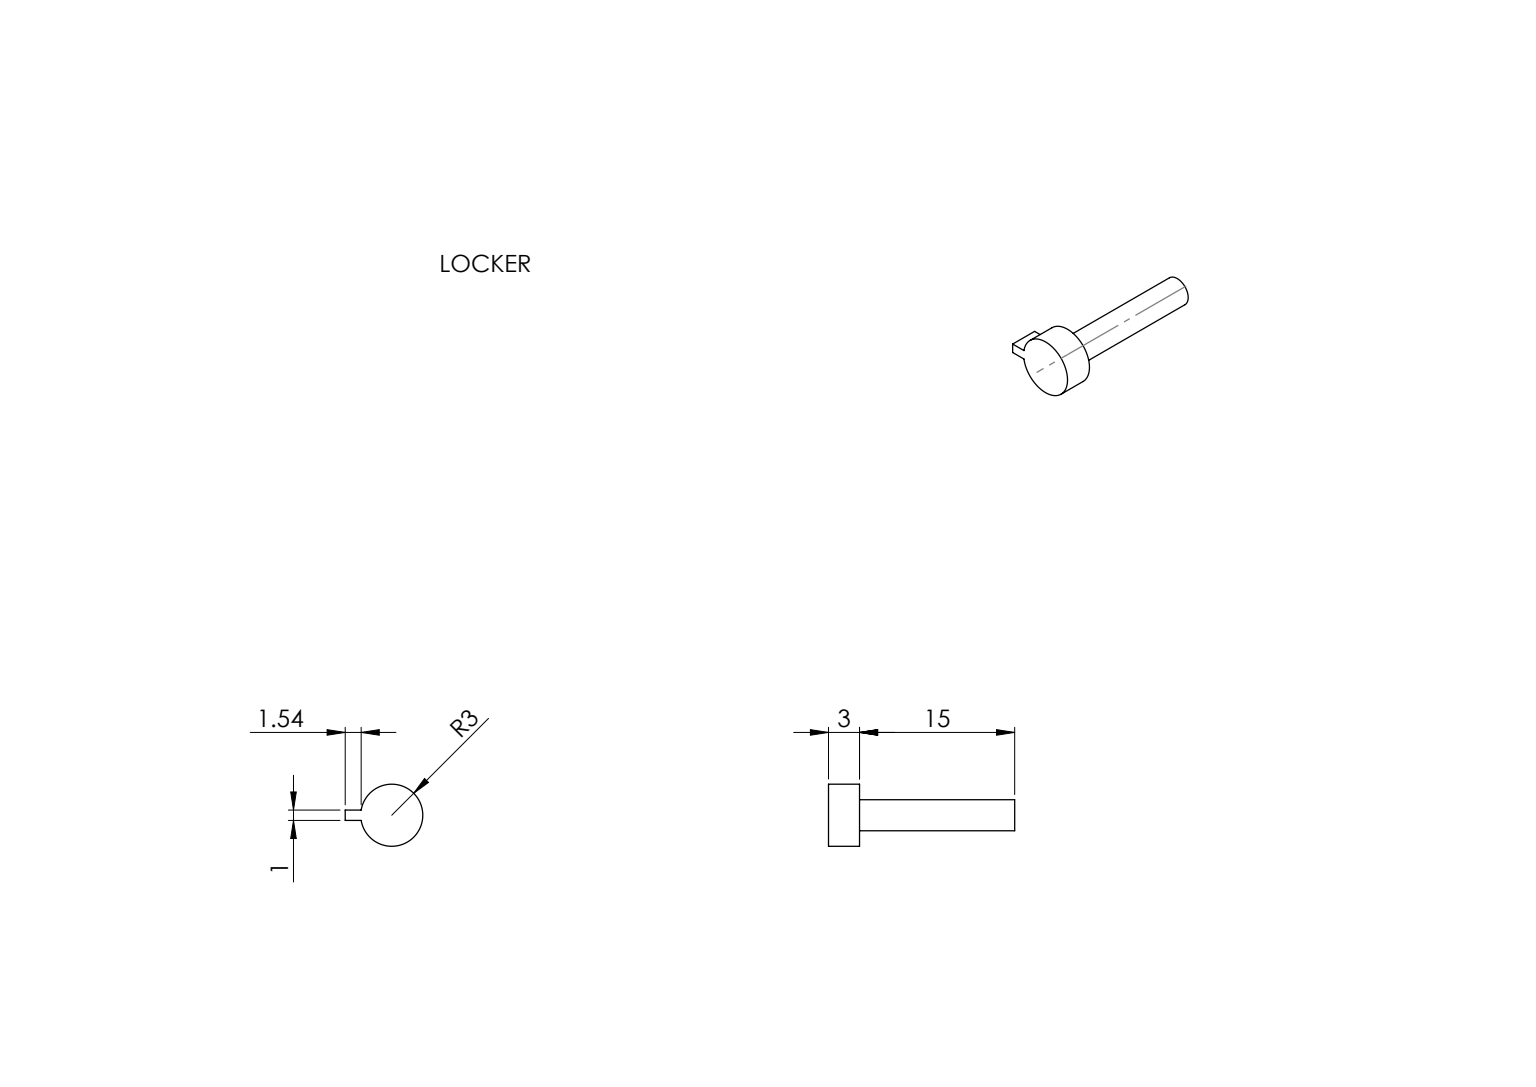
ISO-10303-21;
HEADER;
FILE_DESCRIPTION (('STEP AP214'),
    '1' );
FILE_NAME ('locker.step',
    '2026-10-08T12:30:53',
    ( '' ),
    ( '' ),
    'SwSTEP 2.0',
    'SolidWorks 2026',
    '' );
FILE_SCHEMA (( 'AUTOMOTIVE_DESIGN' ));
ENDSEC;

DATA;
#21=MECHANICAL_DESIGN_GEOMETRIC_PRESENTATION_REPRESENTATION('',(#419),#8834);
#84=LINE ( 'NONE', #11348, #8005 ) ;
#86=ORIENTED_EDGE ( 'NONE', *, *, #7277, .F. ) ;
#98=DIRECTION ( 'NONE',  ( -0.000000000000000000, 0.000000000000000000, 1.000000000000000000 ) ) ;
#220=PRODUCT ( 'locker', 'locker', '', ( #5871 ) ) ;
#374=( LENGTH_UNIT ( ) NAMED_UNIT ( * ) SI_UNIT ( .MILLI., .METRE. ) );
#389=VECTOR ( 'NONE', #4390, 1000.000000000000000 ) ;
#419=STYLED_ITEM ( 'NONE', ( #8733 ), #4375 ) ;
#434=SURFACE_STYLE_USAGE ( .BOTH. , #4112 ) ;
#484=CARTESIAN_POINT ( 'NONE',  ( -4.500000000000000888, 3.903127820947816751E-15, 0.000000000000000000 ) ) ;
#643=DIRECTION ( 'NONE',  ( -1.000000000000000000, -1.445602896647338917E-16, 0.000000000000000000 ) ) ;
#647=ADVANCED_FACE ( 'NONE', ( #2949 ), #10345, .T. ) ;
#766=CYLINDRICAL_SURFACE ( 'NONE', #2507, 1.500000000000000222 ) ;
#773=ORIENTED_EDGE ( 'NONE', *, *, #5743, .F. ) ;
#787=ORIENTED_EDGE ( 'NONE', *, *, #5743, .T. ) ;
#825=EDGE_CURVE ( 'NONE', #4657, #6571, #6084, .T. ) ;
#833=EDGE_CURVE ( 'NONE', #7905, #2790, #10011, .T. ) ;
#987=DIRECTION ( 'NONE',  ( -8.673617379884035472E-16, -1.000000000000000000, 0.000000000000000000 ) ) ;
#1034=CARTESIAN_POINT ( 'NONE',  ( 0.000000000000000000, 0.000000000000000000, 0.000000000000000000 ) ) ;
#1042=PLANE ( 'NONE',  #11528 ) ;
#1047=DIRECTION ( 'NONE',  ( -1.000000000000000000, -1.445602896647339163E-16, 0.000000000000000000 ) ) ;
#1166=CARTESIAN_POINT ( 'NONE',  ( 0.000000000000000000, 0.000000000000000000, 3.000000000000000000 ) ) ;
#1243=FACE_OUTER_BOUND ( 'NONE', #10896, .T. ) ;
#1269=LINE ( 'NONE', #4259, #1726 ) ;
#1297=DIRECTION ( 'NONE',  ( 1.445602896647339163E-16, -1.000000000000000000, 0.000000000000000000 ) ) ;
#1348=ORIENTED_EDGE ( 'NONE', *, *, #833, .F. ) ;
#1393=DIRECTION ( 'NONE',  ( -0.000000000000000000, 0.000000000000000000, 1.000000000000000000 ) ) ;
#1404=DIRECTION ( 'NONE',  ( -0.000000000000000000, -0.000000000000000000, 1.000000000000000000 ) ) ;
#1425=EDGE_CURVE ( 'NONE', #3560, #7905, #5417, .T. ) ;
#1470=ORIENTED_EDGE ( 'NONE', *, *, #3009, .F. ) ;
#1522=ORIENTED_EDGE ( 'NONE', *, *, #6465, .T. ) ;
#1551=DIRECTION ( 'NONE',  ( 0.000000000000000000, 0.000000000000000000, 1.000000000000000000 ) ) ;
#1580=EDGE_LOOP ( 'NONE', ( #3082, #9963, #2261, #1740 ) ) ;
#1644=EDGE_CURVE ( 'NONE', #4353, #2834, #9779, .T. ) ;
#1674=CARTESIAN_POINT ( 'NONE',  ( 0.000000000000000000, 0.000000000000000000, 0.000000000000000000 ) ) ;
#1688=VECTOR ( 'NONE', #1404, 1000.000000000000000 ) ;
#1726=VECTOR ( 'NONE', #5002, 1000.000000000000000 ) ;
#1737=ORIENTED_EDGE ( 'NONE', *, *, #3104, .F. ) ;
#1740=ORIENTED_EDGE ( 'NONE', *, *, #3104, .T. ) ;
#1741=PLANE ( 'NONE',  #6816 ) ;
#1843=ORIENTED_EDGE ( 'NONE', *, *, #3009, .T. ) ;
#1844=CARTESIAN_POINT ( 'NONE',  ( -4.500000000000000888, 3.903127820947816751E-15, 3.000000000000000000 ) ) ;
#1911=CARTESIAN_POINT ( 'NONE',  ( -2.958039891549808953, -0.4999999999999997780, 3.000000000000000000 ) ) ;
#2021=VERTEX_POINT ( 'NONE', #11151 ) ;
#2062=CARTESIAN_POINT ( 'NONE',  ( 0.000000000000000000, 0.000000000000000000, -15.00000000000000000 ) ) ;
#2072=CARTESIAN_POINT ( 'NONE',  ( -4.500000000000000000, 0.4999999999999998890, 3.000000000000000000 ) ) ;
#2077=ORIENTED_EDGE ( 'NONE', *, *, #1425, .F. ) ;
#2096=( NAMED_UNIT ( * ) SI_UNIT ( $, .STERADIAN. ) SOLID_ANGLE_UNIT ( ) );
#2102=ADVANCED_FACE ( 'NONE', ( #10529 ), #3991, .T. ) ;
#2146=DIRECTION ( 'NONE',  ( 1.000000000000000000, 0.000000000000000000, 0.000000000000000000 ) ) ;
#2154=SURFACE_STYLE_FILL_AREA ( #10536 ) ;
#2218=SHAPE_REPRESENTATION_RELATIONSHIP ( 'NONE' , 'NONE' ,  #8353, #2941 ) ;
#2261=ORIENTED_EDGE ( 'NONE', *, *, #1425, .T. ) ;
#2274=DIRECTION ( 'NONE',  ( 1.000000000000000000, 1.445602896647339163E-16, 0.000000000000000000 ) ) ;
#2407=AXIS2_PLACEMENT_3D ( 'NONE', #1034, #98, #3844 ) ;
#2486=DIRECTION ( 'NONE',  ( -1.000000000000000000, 0.000000000000000000, 0.000000000000000000 ) ) ;
#2507=AXIS2_PLACEMENT_3D ( 'NONE', #11053, #10008, #5371 ) ;
#2549=CARTESIAN_POINT ( 'NONE',  ( -4.500000000000000888, -0.5000000000000000000, 3.000000000000000000 ) ) ;
#2653=DIRECTION ( 'NONE',  ( 1.000000000000000000, 0.000000000000000000, 0.000000000000000000 ) ) ;
#2742=LINE ( 'NONE', #2931, #8579 ) ;
#2773=ADVANCED_FACE ( 'NONE', ( #6657 ), #1042, .T. ) ;
#2790=VERTEX_POINT ( 'NONE', #2072 ) ;
#2824=LINE ( 'NONE', #4658, #3000 ) ;
#2834=VERTEX_POINT ( 'NONE', #5988 ) ;
#2887=AXIS2_PLACEMENT_3D ( 'NONE', #9020, #4365, #11365 ) ;
#2931=CARTESIAN_POINT ( 'NONE',  ( -7.228014483236704444E-17, 0.5000000000000005551, 0.000000000000000000 ) ) ;
#2936=ORIENTED_EDGE ( 'NONE', *, *, #5921, .F. ) ;
#2941=ADVANCED_BREP_SHAPE_REPRESENTATION ( '', ( #4375, #8474 ), #5098 ) ;
#2949=FACE_OUTER_BOUND ( 'NONE', #8368, .T. ) ;
#2952=CARTESIAN_POINT ( 'NONE',  ( 0.000000000000000000, 0.000000000000000000, -15.00000000000000000 ) ) ;
#2964=AXIS2_PLACEMENT_3D ( 'NONE', #8180, #3596, #11968 ) ;
#2985=ORIENTED_EDGE ( 'NONE', *, *, #8756, .T. ) ;
#3000=VECTOR ( 'NONE', #1047, 1000.000000000000000 ) ;
#3009=EDGE_CURVE ( 'NONE', #2790, #9956, #9102, .T. ) ;
#3074=ORIENTED_EDGE ( 'NONE', *, *, #6475, .T. ) ;
#3082=ORIENTED_EDGE ( 'NONE', *, *, #6465, .F. ) ;
#3103=CIRCLE ( 'NONE', #8177, 1.500000000000000222 ) ;
#3104=EDGE_CURVE ( 'NONE', #7905, #2021, #84, .T. ) ;
#3111=AXIS2_PLACEMENT_3D ( 'NONE', #3267, #3158, #6876 ) ;
#3158=DIRECTION ( 'NONE',  ( -0.000000000000000000, 0.000000000000000000, 1.000000000000000000 ) ) ;
#3253=PRESENTATION_STYLE_ASSIGNMENT (( #434 ) ) ;
#3267=CARTESIAN_POINT ( 'NONE',  ( 0.000000000000000000, 0.000000000000000000, 3.000000000000000000 ) ) ;
#3361=CARTESIAN_POINT ( 'NONE',  ( 0.000000000000000000, 0.000000000000000000, 0.000000000000000000 ) ) ;
#3515=LINE ( 'NONE', #6332, #6560 ) ;
#3560=VERTEX_POINT ( 'NONE', #1911 ) ;
#3596=DIRECTION ( 'NONE',  ( 0.000000000000000000, 0.000000000000000000, -1.000000000000000000 ) ) ;
#3667=ORIENTED_EDGE ( 'NONE', *, *, #4870, .T. ) ;
#3831=DIRECTION ( 'NONE',  ( -0.000000000000000000, -0.000000000000000000, -1.000000000000000000 ) ) ;
#3844=DIRECTION ( 'NONE',  ( 1.000000000000000000, 0.000000000000000000, 0.000000000000000000 ) ) ;
#3910=DIRECTION ( 'NONE',  ( 1.445602896647338917E-16, -1.000000000000000000, 0.000000000000000000 ) ) ;
#3962=FACE_OUTER_BOUND ( 'NONE', #9270, .T. ) ;
#3984=CARTESIAN_POINT ( 'NONE',  ( -1.500000000000000222, 1.836970198721030181E-16, -15.00000000000000000 ) ) ;
#3985=ORIENTED_EDGE ( 'NONE', *, *, #1644, .T. ) ;
#3991=CYLINDRICAL_SURFACE ( 'NONE', #9791, 1.500000000000000222 ) ;
#4016=SURFACE_STYLE_USAGE ( .BOTH. , #8789 ) ;
#4051=PLANE ( 'NONE',  #8134 ) ;
#4073=( NAMED_UNIT ( * ) SI_UNIT ( $, .STERADIAN. ) SOLID_ANGLE_UNIT ( ) );
#4112=SURFACE_SIDE_STYLE ('',( #2154 ) ) ;
#4159=CIRCLE ( 'NONE', #10407, 1.500000000000000222 ) ;
#4196=FILL_AREA_STYLE_COLOUR ( '', #5502 ) ;
#4259=CARTESIAN_POINT ( 'NONE',  ( 1.500000000000000222, 0.000000000000000000, -15.00000000000000000 ) ) ;
#4353=VERTEX_POINT ( 'NONE', #9237 ) ;
#4365=DIRECTION ( 'NONE',  ( 0.000000000000000000, 0.000000000000000000, -1.000000000000000000 ) ) ;
#4375=MANIFOLD_SOLID_BREP ( 'Boss-Extrude2', #11367 ) ;
#4390=DIRECTION ( 'NONE',  ( -0.000000000000000000, -0.000000000000000000, -1.000000000000000000 ) ) ;
#4430=AXIS2_PLACEMENT_3D ( 'NONE', #6488, #7462, #7525 ) ;
#4472=CIRCLE ( 'NONE', #3111, 3.000000000000000444 ) ;
#4513=ORIENTED_EDGE ( 'NONE', *, *, #9872, .T. ) ;
#4515=COLOUR_RGB ( '', 0.31764706, 0.68627451, 0.89019608) ;
#4580=ORIENTED_EDGE ( 'NONE', *, *, #7558, .F. ) ;
#4597=ORIENTED_EDGE ( 'NONE', *, *, #7558, .T. ) ;
#4603=FACE_OUTER_BOUND ( 'NONE', #6498, .T. ) ;
#4657=VERTEX_POINT ( 'NONE', #4680 ) ;
#4658=CARTESIAN_POINT ( 'NONE',  ( -7.228014483236704444E-17, 0.5000000000000005551, 3.000000000000000000 ) ) ;
#4680=CARTESIAN_POINT ( 'NONE',  ( 1.500000000000000222, 0.000000000000000000, 0.000000000000000000 ) ) ;
#4870=EDGE_CURVE ( 'NONE', #8517, #2790, #2824, .T. ) ;
#4896=AXIS2_PLACEMENT_3D ( 'NONE', #8293, #6453, #6749 ) ;
#4963=LINE ( 'NONE', #3984, #1688 ) ;
#5002=DIRECTION ( 'NONE',  ( -0.000000000000000000, -0.000000000000000000, 1.000000000000000000 ) ) ;
#5098=( GEOMETRIC_REPRESENTATION_CONTEXT ( 3 ) GLOBAL_UNCERTAINTY_ASSIGNED_CONTEXT ( ( #7945 ) ) GLOBAL_UNIT_ASSIGNED_CONTEXT ( ( #374, #9801, #7779 ) ) REPRESENTATION_CONTEXT ( 'NONE', 'WORKASPACE' ) );
#5227=CARTESIAN_POINT ( 'NONE',  ( -2.958039891549808953, -0.4999999999999997780, 0.000000000000000000 ) ) ;
#5284=PLANE ( 'NONE',  #2887 ) ;
#5371=DIRECTION ( 'NONE',  ( 1.000000000000000000, 0.000000000000000000, 0.000000000000000000 ) ) ;
#5417=LINE ( 'NONE', #7178, #7848 ) ;
#5502=COLOUR_RGB ( '', 0.31764706, 0.68627451, 0.89019608) ;
#5612=PRODUCT_DEFINITION ( 'UNKNOWN', '', #6461, #8318 ) ;
#5676=ORIENTED_EDGE ( 'NONE', *, *, #4870, .F. ) ;
#5743=EDGE_CURVE ( 'NONE', #10686, #6311, #8273, .T. ) ;
#5751=DIRECTION ( 'NONE',  ( -1.000000000000000000, -1.445602896647339163E-16, 0.000000000000000000 ) ) ;
#5760=FACE_OUTER_BOUND ( 'NONE', #10530, .T. ) ;
#5786=ORIENTED_EDGE ( 'NONE', *, *, #7277, .T. ) ;
#5814=ORIENTED_EDGE ( 'NONE', *, *, #9278, .T. ) ;
#5871=PRODUCT_CONTEXT ( 'NONE', #7781, 'mechanical' ) ;
#5917=SURFACE_STYLE_FILL_AREA ( #9758 ) ;
#5921=EDGE_CURVE ( 'NONE', #2834, #4353, #4159, .T. ) ;
#5930=DIRECTION ( 'NONE',  ( 1.000000000000000000, 1.445602896647338917E-16, 0.000000000000000000 ) ) ;
#5988=CARTESIAN_POINT ( 'NONE',  ( 1.500000000000000222, 0.000000000000000000, -15.00000000000000000 ) ) ;
#6009=( NAMED_UNIT ( * ) PLANE_ANGLE_UNIT ( ) SI_UNIT ( $, .RADIAN. ) );
#6054=ADVANCED_FACE ( 'NONE', ( #3962 ), #5284, .T. ) ;
#6084=CIRCLE ( 'NONE', #2964, 1.500000000000000222 ) ;
#6122=DIRECTION ( 'NONE',  ( 8.673617379884035472E-16, 1.000000000000000000, 0.000000000000000000 ) ) ;
#6203=DIRECTION ( 'NONE',  ( 0.000000000000000000, 0.000000000000000000, -1.000000000000000000 ) ) ;
#6231=EDGE_LOOP ( 'NONE', ( #86, #2936, #2985, #10305 ) ) ;
#6235=FACE_BOUND ( 'NONE', #10567, .T. ) ;
#6311=VERTEX_POINT ( 'NONE', #6930 ) ;
#6332=CARTESIAN_POINT ( 'NONE',  ( -2.958039891549808509, 0.5000000000000001110, 3.000000000000000000 ) ) ;
#6414=CARTESIAN_POINT ( 'NONE',  ( -2.958039891549808509, 0.5000000000000001110, 3.000000000000000000 ) ) ;
#6453=DIRECTION ( 'NONE',  ( 0.000000000000000000, 0.000000000000000000, -1.000000000000000000 ) ) ;
#6461=PRODUCT_DEFINITION_FORMATION_WITH_SPECIFIED_SOURCE ( 'ANY', '', #220, .NOT_KNOWN. ) ;
#6465=EDGE_CURVE ( 'NONE', #10686, #2021, #11041, .T. ) ;
#6475=EDGE_CURVE ( 'NONE', #8517, #6311, #3515, .T. ) ;
#6488=CARTESIAN_POINT ( 'NONE',  ( 0.000000000000000000, 0.000000000000000000, 3.000000000000000000 ) ) ;
#6498=EDGE_LOOP ( 'NONE', ( #8099, #1737, #6644, #1843 ) ) ;
#6547=ORIENTED_EDGE ( 'NONE', *, *, #5921, .T. ) ;
#6560=VECTOR ( 'NONE', #9993, 1000.000000000000000 ) ;
#6571=VERTEX_POINT ( 'NONE', #11161 ) ;
#6605=CYLINDRICAL_SURFACE ( 'NONE', #4430, 3.000000000000000444 ) ;
#6631=CARTESIAN_POINT ( 'NONE',  ( -4.500000000000000000, 0.4999999999999998890, 3.000000000000000000 ) ) ;
#6644=ORIENTED_EDGE ( 'NONE', *, *, #833, .T. ) ;
#6657=FACE_OUTER_BOUND ( 'NONE', #1580, .T. ) ;
#6749=DIRECTION ( 'NONE',  ( -1.000000000000000000, 0.000000000000000000, 0.000000000000000000 ) ) ;
#6808=ADVANCED_FACE ( 'NONE', ( #1243 ), #4051, .F. ) ;
#6816=AXIS2_PLACEMENT_3D ( 'NONE', #3361, #9214, #10828 ) ;
#6822=DIRECTION ( 'NONE',  ( -1.000000000000000000, 0.000000000000000000, 0.000000000000000000 ) ) ;
#6876=DIRECTION ( 'NONE',  ( 1.000000000000000000, 0.000000000000000000, 0.000000000000000000 ) ) ;
#6930=CARTESIAN_POINT ( 'NONE',  ( -2.958039891549808509, 0.5000000000000001110, 0.000000000000000000 ) ) ;
#7126=ADVANCED_FACE ( 'NONE', ( #5760 ), #6605, .T. ) ;
#7153=CARTESIAN_POINT ( 'NONE',  ( -2.958039891549808953, -0.4999999999999997780, 3.000000000000000000 ) ) ;
#7178=CARTESIAN_POINT ( 'NONE',  ( 7.228014483236684722E-17, -0.4999999999999993339, 3.000000000000000000 ) ) ;
#7277=EDGE_CURVE ( 'NONE', #4353, #6571, #4963, .T. ) ;
#7305=CARTESIAN_POINT ( 'NONE',  ( -4.500000000000000888, 3.903127820947816751E-15, 3.000000000000000000 ) ) ;
#7462=DIRECTION ( 'NONE',  ( -0.000000000000000000, -0.000000000000000000, -1.000000000000000000 ) ) ;
#7525=DIRECTION ( 'NONE',  ( -1.000000000000000000, 0.000000000000000000, 0.000000000000000000 ) ) ;
#7558=EDGE_CURVE ( 'NONE', #6311, #9956, #2742, .T. ) ;
#7631=( GEOMETRIC_REPRESENTATION_CONTEXT ( 3 ) GLOBAL_UNCERTAINTY_ASSIGNED_CONTEXT ( ( #8812 ) ) GLOBAL_UNIT_ASSIGNED_CONTEXT ( ( #7845, #6009, #2096 ) ) REPRESENTATION_CONTEXT ( 'NONE', 'WORKASPACE' ) );
#7771=VECTOR ( 'NONE', #9867, 1000.000000000000000 ) ;
#7779=( NAMED_UNIT ( * ) SI_UNIT ( $, .STERADIAN. ) SOLID_ANGLE_UNIT ( ) );
#7781=APPLICATION_CONTEXT ( 'automotive_design' ) ;
#7845=( LENGTH_UNIT ( ) NAMED_UNIT ( * ) SI_UNIT ( .MILLI., .METRE. ) );
#7848=VECTOR ( 'NONE', #643, 1000.000000000000000 ) ;
#7905=VERTEX_POINT ( 'NONE', #2549 ) ;
#7945=UNCERTAINTY_MEASURE_WITH_UNIT (LENGTH_MEASURE( 1.000000000000000082E-05 ), #374, 'distance_accuracy_value', 'NONE');
#8005=VECTOR ( 'NONE', #3831, 1000.000000000000000 ) ;
#8009=APPLICATION_CONTEXT ( 'automotive_design' ) ;
#8099=ORIENTED_EDGE ( 'NONE', *, *, #11699, .F. ) ;
#8134=AXIS2_PLACEMENT_3D ( 'NONE', #11516, #1297, #2274 ) ;
#8177=AXIS2_PLACEMENT_3D ( 'NONE', #10875, #8918, #2486 ) ;
#8180=CARTESIAN_POINT ( 'NONE',  ( 0.000000000000000000, 0.000000000000000000, 0.000000000000000000 ) ) ;
#8208=CARTESIAN_POINT ( 'NONE',  ( -4.500000000000000000, 0.4999999999999998890, 0.000000000000000000 ) ) ;
#8236=ORIENTED_EDGE ( 'NONE', *, *, #9278, .F. ) ;
#8273=CIRCLE ( 'NONE', #2407, 3.000000000000000444 ) ;
#8293=CARTESIAN_POINT ( 'NONE',  ( 0.000000000000000000, 0.000000000000000000, -15.00000000000000000 ) ) ;
#8318=PRODUCT_DEFINITION_CONTEXT ( 'detailed design', #8009, 'design' ) ;
#8347=DIRECTION ( 'NONE',  ( -1.000000000000000000, -1.445602896647338917E-16, 0.000000000000000000 ) ) ;
#8353=SHAPE_REPRESENTATION ( 'locker', ( #8474 ), #5098 ) ;
#8368=EDGE_LOOP ( 'NONE', ( #5814, #3667, #1348, #2077 ) ) ;
#8392=ORIENTED_EDGE ( 'NONE', *, *, #8754, .F. ) ;
#8393=ADVANCED_FACE ( 'NONE', ( #6235, #11737 ), #1741, .F. ) ;
#8395=DIRECTION ( 'NONE',  ( -1.000000000000000000, 8.673617379884035472E-16, 0.000000000000000000 ) ) ;
#8450=( NAMED_UNIT ( * ) PLANE_ANGLE_UNIT ( ) SI_UNIT ( $, .RADIAN. ) );
#8463=AXIS2_PLACEMENT_3D ( 'NONE', #1166, #1393, #11393 ) ;
#8474=AXIS2_PLACEMENT_3D ( 'NONE', #1674, #1551, #2653 ) ;
#8517=VERTEX_POINT ( 'NONE', #6414 ) ;
#8579=VECTOR ( 'NONE', #5751, 1000.000000000000000 ) ;
#8674=( LENGTH_UNIT ( ) NAMED_UNIT ( * ) SI_UNIT ( .MILLI., .METRE. ) );
#8694=SHAPE_DEFINITION_REPRESENTATION ( #10490, #8353 ) ;
#8733=PRESENTATION_STYLE_ASSIGNMENT (( #4016 ) ) ;
#8754=EDGE_CURVE ( 'NONE', #6571, #4657, #3103, .T. ) ;
#8756=EDGE_CURVE ( 'NONE', #2834, #4657, #1269, .T. ) ;
#8761=DIRECTION ( 'NONE',  ( -0.000000000000000000, -0.000000000000000000, 1.000000000000000000 ) ) ;
#8768=FILL_AREA_STYLE_COLOUR ( '', #4515 ) ;
#8789=SURFACE_SIDE_STYLE ('',( #5917 ) ) ;
#8812=UNCERTAINTY_MEASURE_WITH_UNIT (LENGTH_MEASURE( 1.000000000000000082E-05 ), #7845, 'distance_accuracy_value', 'NONE');
#8834=( GEOMETRIC_REPRESENTATION_CONTEXT ( 3 ) GLOBAL_UNCERTAINTY_ASSIGNED_CONTEXT ( ( #11855 ) ) GLOBAL_UNIT_ASSIGNED_CONTEXT ( ( #8674, #8450, #4073 ) ) REPRESENTATION_CONTEXT ( 'NONE', 'WORKASPACE' ) );
#8880=LINE ( 'NONE', #484, #11957 ) ;
#8910=ADVANCED_FACE ( 'NONE', ( #10931 ), #766, .T. ) ;
#8918=DIRECTION ( 'NONE',  ( 0.000000000000000000, 0.000000000000000000, -1.000000000000000000 ) ) ;
#9020=CARTESIAN_POINT ( 'NONE',  ( 0.000000000000000000, 0.000000000000000000, -15.00000000000000000 ) ) ;
#9102=LINE ( 'NONE', #6631, #389 ) ;
#9192=CARTESIAN_POINT ( 'NONE',  ( 7.228014483236684722E-17, -0.4999999999999993339, 0.000000000000000000 ) ) ;
#9211=VECTOR ( 'NONE', #10879, 1000.000000000000000 ) ;
#9214=DIRECTION ( 'NONE',  ( -0.000000000000000000, 0.000000000000000000, 1.000000000000000000 ) ) ;
#9237=CARTESIAN_POINT ( 'NONE',  ( -1.500000000000000222, 1.836970198721030181E-16, -15.00000000000000000 ) ) ;
#9270=EDGE_LOOP ( 'NONE', ( #6547, #3985 ) ) ;
#9278=EDGE_CURVE ( 'NONE', #3560, #8517, #4472, .T. ) ;
#9487=PLANE ( 'NONE',  #11006 ) ;
#9758=FILL_AREA_STYLE ('',( #4196 ) ) ;
#9779=CIRCLE ( 'NONE', #4896, 1.500000000000000222 ) ;
#9786=STYLED_ITEM ( 'NONE', ( #3253 ), #2941 ) ;
#9791=AXIS2_PLACEMENT_3D ( 'NONE', #2952, #8761, #2146 ) ;
#9801=( NAMED_UNIT ( * ) PLANE_ANGLE_UNIT ( ) SI_UNIT ( $, .RADIAN. ) );
#9867=DIRECTION ( 'NONE',  ( -0.000000000000000000, -0.000000000000000000, -1.000000000000000000 ) ) ;
#9872=EDGE_CURVE ( 'NONE', #3560, #10686, #10901, .T. ) ;
#9900=ORIENTED_EDGE ( 'NONE', *, *, #1644, .F. ) ;
#9956=VERTEX_POINT ( 'NONE', #8208 ) ;
#9963=ORIENTED_EDGE ( 'NONE', *, *, #9872, .F. ) ;
#9993=DIRECTION ( 'NONE',  ( -0.000000000000000000, -0.000000000000000000, -1.000000000000000000 ) ) ;
#10008=DIRECTION ( 'NONE',  ( -0.000000000000000000, -0.000000000000000000, 1.000000000000000000 ) ) ;
#10011=LINE ( 'NONE', #7305, #9211 ) ;
#10039=ADVANCED_FACE ( 'NONE', ( #4603 ), #9487, .T. ) ;
#10065=ORIENTED_EDGE ( 'NONE', *, *, #6475, .F. ) ;
#10172=ORIENTED_EDGE ( 'NONE', *, *, #8756, .F. ) ;
#10305=ORIENTED_EDGE ( 'NONE', *, *, #825, .T. ) ;
#10336=EDGE_LOOP ( 'NONE', ( #773, #1522, #11331, #4580 ) ) ;
#10345=PLANE ( 'NONE',  #8463 ) ;
#10396=CARTESIAN_POINT ( 'NONE',  ( 7.228014483236684722E-17, -0.4999999999999993339, 3.000000000000000000 ) ) ;
#10407=AXIS2_PLACEMENT_3D ( 'NONE', #2062, #6203, #6822 ) ;
#10490=PRODUCT_DEFINITION_SHAPE ( 'NONE', 'NONE',  #5612 ) ;
#10529=FACE_OUTER_BOUND ( 'NONE', #6231, .T. ) ;
#10530=EDGE_LOOP ( 'NONE', ( #787, #10065, #8236, #4513 ) ) ;
#10536=FILL_AREA_STYLE ('',( #8768 ) ) ;
#10567=EDGE_LOOP ( 'NONE', ( #10990, #8392 ) ) ;
#10686=VERTEX_POINT ( 'NONE', #5227 ) ;
#10828=DIRECTION ( 'NONE',  ( 1.000000000000000000, 0.000000000000000000, 0.000000000000000000 ) ) ;
#10875=CARTESIAN_POINT ( 'NONE',  ( 0.000000000000000000, 0.000000000000000000, 0.000000000000000000 ) ) ;
#10879=DIRECTION ( 'NONE',  ( 8.673617379884035472E-16, 1.000000000000000000, 0.000000000000000000 ) ) ;
#10896=EDGE_LOOP ( 'NONE', ( #4597, #1470, #5676, #3074 ) ) ;
#10901=LINE ( 'NONE', #7153, #7771 ) ;
#10931=FACE_OUTER_BOUND ( 'NONE', #11959, .T. ) ;
#10990=ORIENTED_EDGE ( 'NONE', *, *, #825, .F. ) ;
#11006=AXIS2_PLACEMENT_3D ( 'NONE', #1844, #8395, #987 ) ;
#11041=LINE ( 'NONE', #9192, #11835 ) ;
#11053=CARTESIAN_POINT ( 'NONE',  ( 0.000000000000000000, 0.000000000000000000, -15.00000000000000000 ) ) ;
#11151=CARTESIAN_POINT ( 'NONE',  ( -4.500000000000000888, -0.5000000000000000000, 0.000000000000000000 ) ) ;
#11158=MECHANICAL_DESIGN_GEOMETRIC_PRESENTATION_REPRESENTATION('',(#9786),#7631);
#11161=CARTESIAN_POINT ( 'NONE',  ( -1.500000000000000222, 1.836970198721030181E-16, 0.000000000000000000 ) ) ;
#11331=ORIENTED_EDGE ( 'NONE', *, *, #11699, .T. ) ;
#11348=CARTESIAN_POINT ( 'NONE',  ( -4.500000000000000888, -0.5000000000000000000, 3.000000000000000000 ) ) ;
#11365=DIRECTION ( 'NONE',  ( -1.000000000000000000, 0.000000000000000000, -0.000000000000000000 ) ) ;
#11367=CLOSED_SHELL ( 'NONE', ( #8910, #7126, #6808, #10039, #2773, #647, #8393, #2102, #6054 ) ) ;
#11393=DIRECTION ( 'NONE',  ( 1.000000000000000000, 0.000000000000000000, 0.000000000000000000 ) ) ;
#11516=CARTESIAN_POINT ( 'NONE',  ( -7.228014483236704444E-17, 0.5000000000000005551, 3.000000000000000000 ) ) ;
#11528=AXIS2_PLACEMENT_3D ( 'NONE', #10396, #3910, #5930 ) ;
#11699=EDGE_CURVE ( 'NONE', #2021, #9956, #8880, .T. ) ;
#11737=FACE_OUTER_BOUND ( 'NONE', #10336, .T. ) ;
#11835=VECTOR ( 'NONE', #8347, 1000.000000000000000 ) ;
#11855=UNCERTAINTY_MEASURE_WITH_UNIT (LENGTH_MEASURE( 1.000000000000000082E-05 ), #8674, 'distance_accuracy_value', 'NONE');
#11957=VECTOR ( 'NONE', #6122, 1000.000000000000000 ) ;
#11959=EDGE_LOOP ( 'NONE', ( #9900, #5786, #11988, #10172 ) ) ;
#11968=DIRECTION ( 'NONE',  ( -1.000000000000000000, 0.000000000000000000, 0.000000000000000000 ) ) ;
#11988=ORIENTED_EDGE ( 'NONE', *, *, #8754, .T. ) ;
ENDSEC;
END-ISO-10303-21;
